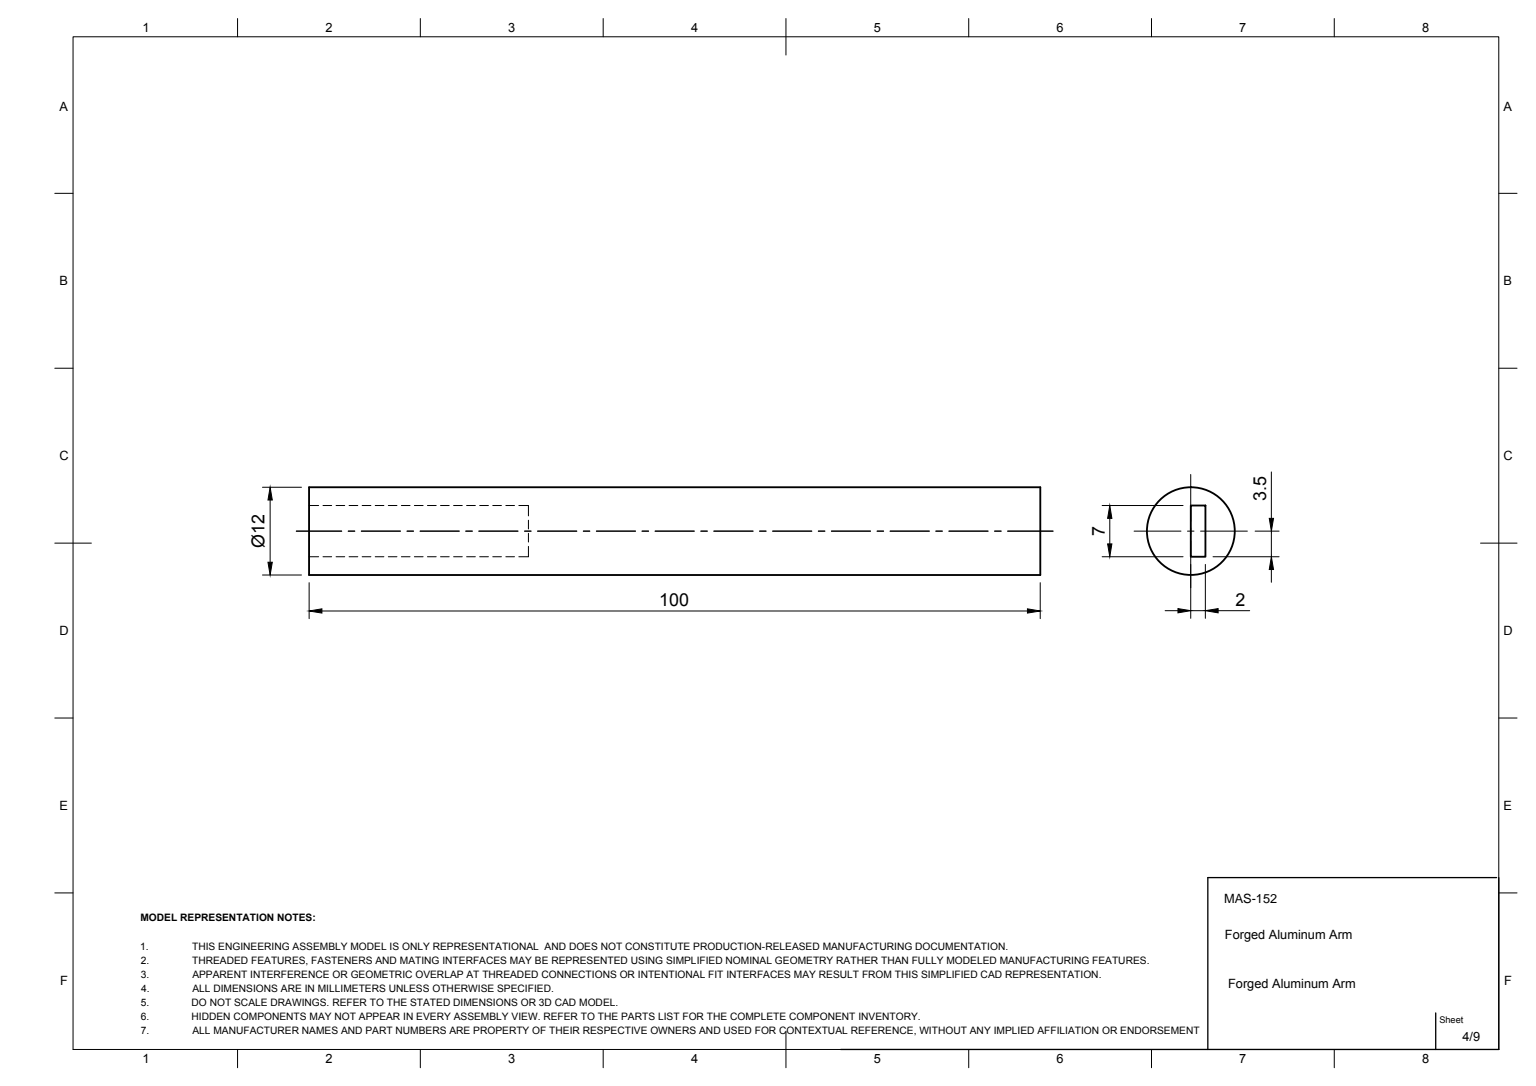
ISO-10303-21;
HEADER;
/* Generated by software containing ST-Developer
 * from STEP Tools, Inc. (www.steptools.com) 
 */

FILE_DESCRIPTION(
/* description */ ('STEP AP214'),
/* implementation_level */ '2;1');

FILE_NAME(
/* name */ 'Forged Aluminum Arm.step',
/* time_stamp */ '2026-11-04T19:18:53-08:00',
/* author */ (''),
/* organization */ (''),
/* preprocessor_version */ 'ST-DEVELOPER v20.2',
/* originating_system */ 'Autodesk Translation Framework v15.17.0.0',
/* authorisation */ '');

FILE_SCHEMA (('AUTOMOTIVE_DESIGN { 1 0 10303 214 3 1 1 }'));
ENDSEC;

DATA;
#10=MECHANICAL_DESIGN_GEOMETRIC_PRESENTATION_REPRESENTATION('',(#82),#5942);
#68=SHAPE_REPRESENTATION_RELATIONSHIP('SRR','None',#5979,#75);
#75=ADVANCED_BREP_SHAPE_REPRESENTATION('',(#89),#5939);
#82=STYLED_ITEM('',(#6022),#89);
#89=MANIFOLD_SOLID_BREP('Body1',#929);
#96=FACE_BOUND('',#233,.T.);
#122=PLANE('',#1071);
#123=PLANE('',#1072);
#124=PLANE('',#1073);
#125=PLANE('',#1074);
#126=PLANE('',#1075);
#127=PLANE('',#1076);
#128=PLANE('',#1077);
#172=FACE_OUTER_BOUND('',#230,.T.);
#173=FACE_OUTER_BOUND('',#231,.T.);
#174=FACE_OUTER_BOUND('',#232,.T.);
#175=FACE_OUTER_BOUND('',#234,.T.);
#176=FACE_OUTER_BOUND('',#235,.T.);
#177=FACE_OUTER_BOUND('',#236,.T.);
#178=FACE_OUTER_BOUND('',#237,.T.);
#179=FACE_OUTER_BOUND('',#238,.T.);
#230=EDGE_LOOP('',(#778,#779,#780,#781));
#231=EDGE_LOOP('',(#782));
#232=EDGE_LOOP('',(#783));
#233=EDGE_LOOP('',(#784,#785,#786,#787));
#234=EDGE_LOOP('',(#788,#789,#790,#791));
#235=EDGE_LOOP('',(#792,#793,#794,#795));
#236=EDGE_LOOP('',(#796,#797,#798,#799));
#237=EDGE_LOOP('',(#800,#801,#802,#803));
#238=EDGE_LOOP('',(#804,#805,#806,#807));
#300=LINE('',#5824,#378);
#301=LINE('',#5830,#379);
#302=LINE('',#5832,#380);
#303=LINE('',#5834,#381);
#304=LINE('',#5835,#382);
#305=LINE('',#5838,#383);
#306=LINE('',#5840,#384);
#307=LINE('',#5841,#385);
#308=LINE('',#5844,#386);
#309=LINE('',#5845,#387);
#310=LINE('',#5848,#388);
#311=LINE('',#5849,#389);
#312=LINE('',#5851,#390);
#378=VECTOR('',#1275,6.);
#379=VECTOR('',#1282,1000.);
#380=VECTOR('',#1283,1000.);
#381=VECTOR('',#1284,1000.);
#382=VECTOR('',#1285,1000.);
#383=VECTOR('',#1288,1000.);
#384=VECTOR('',#1289,1000.);
#385=VECTOR('',#1290,1000.);
#386=VECTOR('',#1293,1000.);
#387=VECTOR('',#1294,1000.);
#388=VECTOR('',#1297,1000.);
#389=VECTOR('',#1298,1000.);
#390=VECTOR('',#1301,1000.);
#436=CIRCLE('',#1069,6.);
#437=CIRCLE('',#1070,6.);
#492=VERTEX_POINT('',#5821);
#493=VERTEX_POINT('',#5823);
#494=VERTEX_POINT('',#5828);
#495=VERTEX_POINT('',#5829);
#496=VERTEX_POINT('',#5831);
#497=VERTEX_POINT('',#5833);
#498=VERTEX_POINT('',#5837);
#499=VERTEX_POINT('',#5839);
#500=VERTEX_POINT('',#5843);
#501=VERTEX_POINT('',#5847);
#592=EDGE_CURVE('',#492,#492,#436,.T.);
#593=EDGE_CURVE('',#492,#493,#300,.T.);
#594=EDGE_CURVE('',#493,#493,#437,.T.);
#595=EDGE_CURVE('',#494,#495,#301,.T.);
#596=EDGE_CURVE('',#494,#496,#302,.T.);
#597=EDGE_CURVE('',#496,#497,#303,.T.);
#598=EDGE_CURVE('',#497,#495,#304,.T.);
#599=EDGE_CURVE('',#494,#498,#305,.T.);
#600=EDGE_CURVE('',#499,#498,#306,.T.);
#601=EDGE_CURVE('',#496,#499,#307,.T.);
#602=EDGE_CURVE('',#500,#495,#308,.T.);
#603=EDGE_CURVE('',#498,#500,#309,.T.);
#604=EDGE_CURVE('',#499,#501,#310,.T.);
#605=EDGE_CURVE('',#501,#497,#311,.T.);
#606=EDGE_CURVE('',#501,#500,#312,.T.);
#778=ORIENTED_EDGE('',*,*,#592,.F.);
#779=ORIENTED_EDGE('',*,*,#593,.T.);
#780=ORIENTED_EDGE('',*,*,#594,.T.);
#781=ORIENTED_EDGE('',*,*,#593,.F.);
#782=ORIENTED_EDGE('',*,*,#592,.T.);
#783=ORIENTED_EDGE('',*,*,#594,.F.);
#784=ORIENTED_EDGE('',*,*,#595,.F.);
#785=ORIENTED_EDGE('',*,*,#596,.T.);
#786=ORIENTED_EDGE('',*,*,#597,.T.);
#787=ORIENTED_EDGE('',*,*,#598,.T.);
#788=ORIENTED_EDGE('',*,*,#599,.T.);
#789=ORIENTED_EDGE('',*,*,#600,.F.);
#790=ORIENTED_EDGE('',*,*,#601,.F.);
#791=ORIENTED_EDGE('',*,*,#596,.F.);
#792=ORIENTED_EDGE('',*,*,#595,.T.);
#793=ORIENTED_EDGE('',*,*,#602,.F.);
#794=ORIENTED_EDGE('',*,*,#603,.F.);
#795=ORIENTED_EDGE('',*,*,#599,.F.);
#796=ORIENTED_EDGE('',*,*,#601,.T.);
#797=ORIENTED_EDGE('',*,*,#604,.T.);
#798=ORIENTED_EDGE('',*,*,#605,.T.);
#799=ORIENTED_EDGE('',*,*,#597,.F.);
#800=ORIENTED_EDGE('',*,*,#605,.F.);
#801=ORIENTED_EDGE('',*,*,#606,.T.);
#802=ORIENTED_EDGE('',*,*,#602,.T.);
#803=ORIENTED_EDGE('',*,*,#598,.F.);
#804=ORIENTED_EDGE('',*,*,#603,.T.);
#805=ORIENTED_EDGE('',*,*,#606,.F.);
#806=ORIENTED_EDGE('',*,*,#604,.F.);
#807=ORIENTED_EDGE('',*,*,#600,.T.);
#867=CYLINDRICAL_SURFACE('',#1068,6.);
#903=ADVANCED_FACE('',(#172),#867,.T.);
#904=ADVANCED_FACE('',(#173),#122,.T.);
#905=ADVANCED_FACE('',(#174,#96),#123,.F.);
#906=ADVANCED_FACE('',(#175),#124,.F.);
#907=ADVANCED_FACE('',(#176),#125,.T.);
#908=ADVANCED_FACE('',(#177),#126,.F.);
#909=ADVANCED_FACE('',(#178),#127,.F.);
#910=ADVANCED_FACE('',(#179),#128,.F.);
#929=CLOSED_SHELL('',(#903,#904,#905,#906,#907,#908,#909,#910));
#1067=AXIS2_PLACEMENT_3D('',#5819,#1269,#1270);
#1068=AXIS2_PLACEMENT_3D('',#5820,#1271,#1272);
#1069=AXIS2_PLACEMENT_3D('',#5822,#1273,#1274);
#1070=AXIS2_PLACEMENT_3D('',#5825,#1276,#1277);
#1071=AXIS2_PLACEMENT_3D('',#5826,#1278,#1279);
#1072=AXIS2_PLACEMENT_3D('',#5827,#1280,#1281);
#1073=AXIS2_PLACEMENT_3D('',#5836,#1286,#1287);
#1074=AXIS2_PLACEMENT_3D('',#5842,#1291,#1292);
#1075=AXIS2_PLACEMENT_3D('',#5846,#1295,#1296);
#1076=AXIS2_PLACEMENT_3D('',#5850,#1299,#1300);
#1077=AXIS2_PLACEMENT_3D('',#5852,#1302,#1303);
#1269=DIRECTION('axis',(0.,0.,1.));
#1270=DIRECTION('refdir',(1.,0.,0.));
#1271=DIRECTION('center_axis',(1.04083408558608E-16,-1.,0.));
#1272=DIRECTION('ref_axis',(1.,1.04083408558608E-16,0.));
#1273=DIRECTION('center_axis',(1.04083408558608E-16,-1.,0.));
#1274=DIRECTION('ref_axis',(1.,1.04083408558608E-16,0.));
#1275=DIRECTION('',(-1.04083408558608E-16,1.,0.));
#1276=DIRECTION('center_axis',(1.04083408558608E-16,-1.,0.));
#1277=DIRECTION('ref_axis',(1.,1.04083408558608E-16,0.));
#1278=DIRECTION('center_axis',(1.04083408558608E-16,-1.,0.));
#1279=DIRECTION('ref_axis',(1.,1.04083408558608E-16,0.));
#1280=DIRECTION('center_axis',(1.04083408558608E-16,-1.,0.));
#1281=DIRECTION('ref_axis',(1.,1.04083408558608E-16,0.));
#1282=DIRECTION('',(1.,1.04083408558608E-16,0.));
#1283=DIRECTION('',(0.,0.,-1.));
#1284=DIRECTION('',(1.,1.04083408558608E-16,0.));
#1285=DIRECTION('',(0.,0.,1.));
#1286=DIRECTION('center_axis',(-1.,-1.51313062618285E-16,0.));
#1287=DIRECTION('ref_axis',(1.51313062618285E-16,-1.,0.));
#1288=DIRECTION('',(1.51313062618285E-16,-1.,0.));
#1289=DIRECTION('',(0.,0.,1.));
#1290=DIRECTION('',(1.51313062618285E-16,-1.,0.));
#1291=DIRECTION('center_axis',(0.,0.,-1.));
#1292=DIRECTION('ref_axis',(-1.,0.,0.));
#1293=DIRECTION('',(-6.93889390390723E-17,1.,0.));
#1294=DIRECTION('',(1.,0.,0.));
#1295=DIRECTION('center_axis',(0.,0.,-1.));
#1296=DIRECTION('ref_axis',(-1.,0.,0.));
#1297=DIRECTION('',(1.,0.,0.));
#1298=DIRECTION('',(-6.93889390390723E-17,1.,0.));
#1299=DIRECTION('center_axis',(1.,6.93889390390723E-17,0.));
#1300=DIRECTION('ref_axis',(-6.93889390390723E-17,1.,0.));
#1301=DIRECTION('',(0.,0.,1.));
#1302=DIRECTION('center_axis',(0.,-1.,0.));
#1303=DIRECTION('ref_axis',(0.,0.,-1.));
#5819=CARTESIAN_POINT('',(0.,0.,0.));
#5820=CARTESIAN_POINT('Origin',(15.6421356237309,-34.142135623731,0.));
#5821=CARTESIAN_POINT('',(9.64213562373089,-134.142135623731,-7.34788079488412E-16));
#5822=CARTESIAN_POINT('Origin',(15.6421356237309,-134.142135623731,0.));
#5823=CARTESIAN_POINT('',(9.64213562373088,-34.142135623731,-7.34788079488412E-16));
#5824=CARTESIAN_POINT('',(9.64213562373088,-34.142135623731,-7.34788079488412E-16));
#5825=CARTESIAN_POINT('Origin',(15.6421356237309,-34.142135623731,0.));
#5826=CARTESIAN_POINT('Origin',(15.6421356237309,-134.142135623731,0.));
#5827=CARTESIAN_POINT('Origin',(15.6421356237309,-34.142135623731,0.));
#5828=CARTESIAN_POINT('',(12.1421356237309,-34.142135623731,2.));
#5829=CARTESIAN_POINT('',(19.1421356237309,-34.142135623731,2.));
#5830=CARTESIAN_POINT('',(15.6421356237309,-34.142135623731,2.));
#5831=CARTESIAN_POINT('',(12.1421356237309,-34.142135623731,0.));
#5832=CARTESIAN_POINT('',(12.1421356237309,-34.142135623731,0.));
#5833=CARTESIAN_POINT('',(19.1421356237309,-34.142135623731,0.));
#5834=CARTESIAN_POINT('',(15.6421356237309,-34.142135623731,0.));
#5835=CARTESIAN_POINT('',(19.1421356237309,-34.142135623731,0.));
#5836=CARTESIAN_POINT('Origin',(12.1421356237309,-18.2842712474619,0.));
#5837=CARTESIAN_POINT('',(12.1421356237309,-64.142135623731,2.));
#5838=CARTESIAN_POINT('',(12.1421356237309,-18.2842712474619,2.));
#5839=CARTESIAN_POINT('',(12.1421356237309,-64.142135623731,0.));
#5840=CARTESIAN_POINT('',(12.1421356237309,-64.142135623731,0.));
#5841=CARTESIAN_POINT('',(12.1421356237309,-18.2842712474619,0.));
#5842=CARTESIAN_POINT('Origin',(0.,0.,2.));
#5843=CARTESIAN_POINT('',(19.1421356237309,-64.142135623731,2.));
#5844=CARTESIAN_POINT('',(19.1421356237309,-14.142135623731,2.));
#5845=CARTESIAN_POINT('',(9.14213562373088,-64.142135623731,2.));
#5846=CARTESIAN_POINT('Origin',(0.,0.,0.));
#5847=CARTESIAN_POINT('',(19.1421356237309,-64.142135623731,0.));
#5848=CARTESIAN_POINT('',(9.14213562373088,-64.142135623731,0.));
#5849=CARTESIAN_POINT('',(19.1421356237309,-14.142135623731,0.));
#5850=CARTESIAN_POINT('Origin',(19.1421356237309,-14.142135623731,0.));
#5851=CARTESIAN_POINT('',(19.1421356237309,-64.142135623731,0.));
#5852=CARTESIAN_POINT('Origin',(9.14213562373088,-64.142135623731,0.));
#5930=UNCERTAINTY_MEASURE_WITH_UNIT(LENGTH_MEASURE(0.01),#5943,
'DISTANCE_ACCURACY_VALUE',
'Maximum model space distance between geometric entities at asserted c
onnectivities');
#5933=UNCERTAINTY_MEASURE_WITH_UNIT(LENGTH_MEASURE(0.01),#5943,
'DISTANCE_ACCURACY_VALUE',
'Maximum model space distance between geometric entities at asserted c
onnectivities');
#5939=(
GEOMETRIC_REPRESENTATION_CONTEXT(3)
GLOBAL_UNCERTAINTY_ASSIGNED_CONTEXT((#5930))
GLOBAL_UNIT_ASSIGNED_CONTEXT((#5943,#5945,#5946))
REPRESENTATION_CONTEXT('','3D')
);
#5942=(
GEOMETRIC_REPRESENTATION_CONTEXT(3)
GLOBAL_UNCERTAINTY_ASSIGNED_CONTEXT((#5933))
GLOBAL_UNIT_ASSIGNED_CONTEXT((#5943,#5945,#5946))
REPRESENTATION_CONTEXT('','3D')
);
#5943=(
LENGTH_UNIT()
NAMED_UNIT(*)
SI_UNIT(.MILLI.,.METRE.)
);
#5945=(
NAMED_UNIT(*)
PLANE_ANGLE_UNIT()
SI_UNIT($,.RADIAN.)
);
#5946=(
NAMED_UNIT(*)
SI_UNIT($,.STERADIAN.)
SOLID_ANGLE_UNIT()
);
#5952=SHAPE_DEFINITION_REPRESENTATION(#5960,#5979);
#5960=PRODUCT_DEFINITION_SHAPE('',$,#5988);
#5979=SHAPE_REPRESENTATION('',(#1067),#5939);
#5982=PRODUCT_DEFINITION_CONTEXT('part definition',#6008,'design');
#5988=PRODUCT_DEFINITION('Forged Aluminum Arm','Forged Aluminum Arm',#5996,
#5982);
#5996=PRODUCT_DEFINITION_FORMATION('',$,#6015);
#6008=APPLICATION_CONTEXT(
'Core Data for Automotive Mechanical Design Process');
#6009=PRODUCT_CONTEXT('part definition',#6008,'mechanical');
#6015=PRODUCT('Forged Aluminum Arm','Forged Aluminum Arm',$,(#6009));
#6022=PRESENTATION_STYLE_ASSIGNMENT((#6028));
#6028=SURFACE_STYLE_USAGE(.BOTH.,#6034);
#6034=SURFACE_SIDE_STYLE('',(#6040));
#6040=SURFACE_STYLE_FILL_AREA(#6046);
#6046=FILL_AREA_STYLE('Opaque(97,158,199)',(#6052));
#6052=FILL_AREA_STYLE_COLOUR('Opaque(97,158,199)',#6058);
#6058=COLOUR_RGB('Opaque(97,158,199)',0.380392156862745,0.619607843137255,
0.780392156862745);
ENDSEC;
END-ISO-10303-21;
